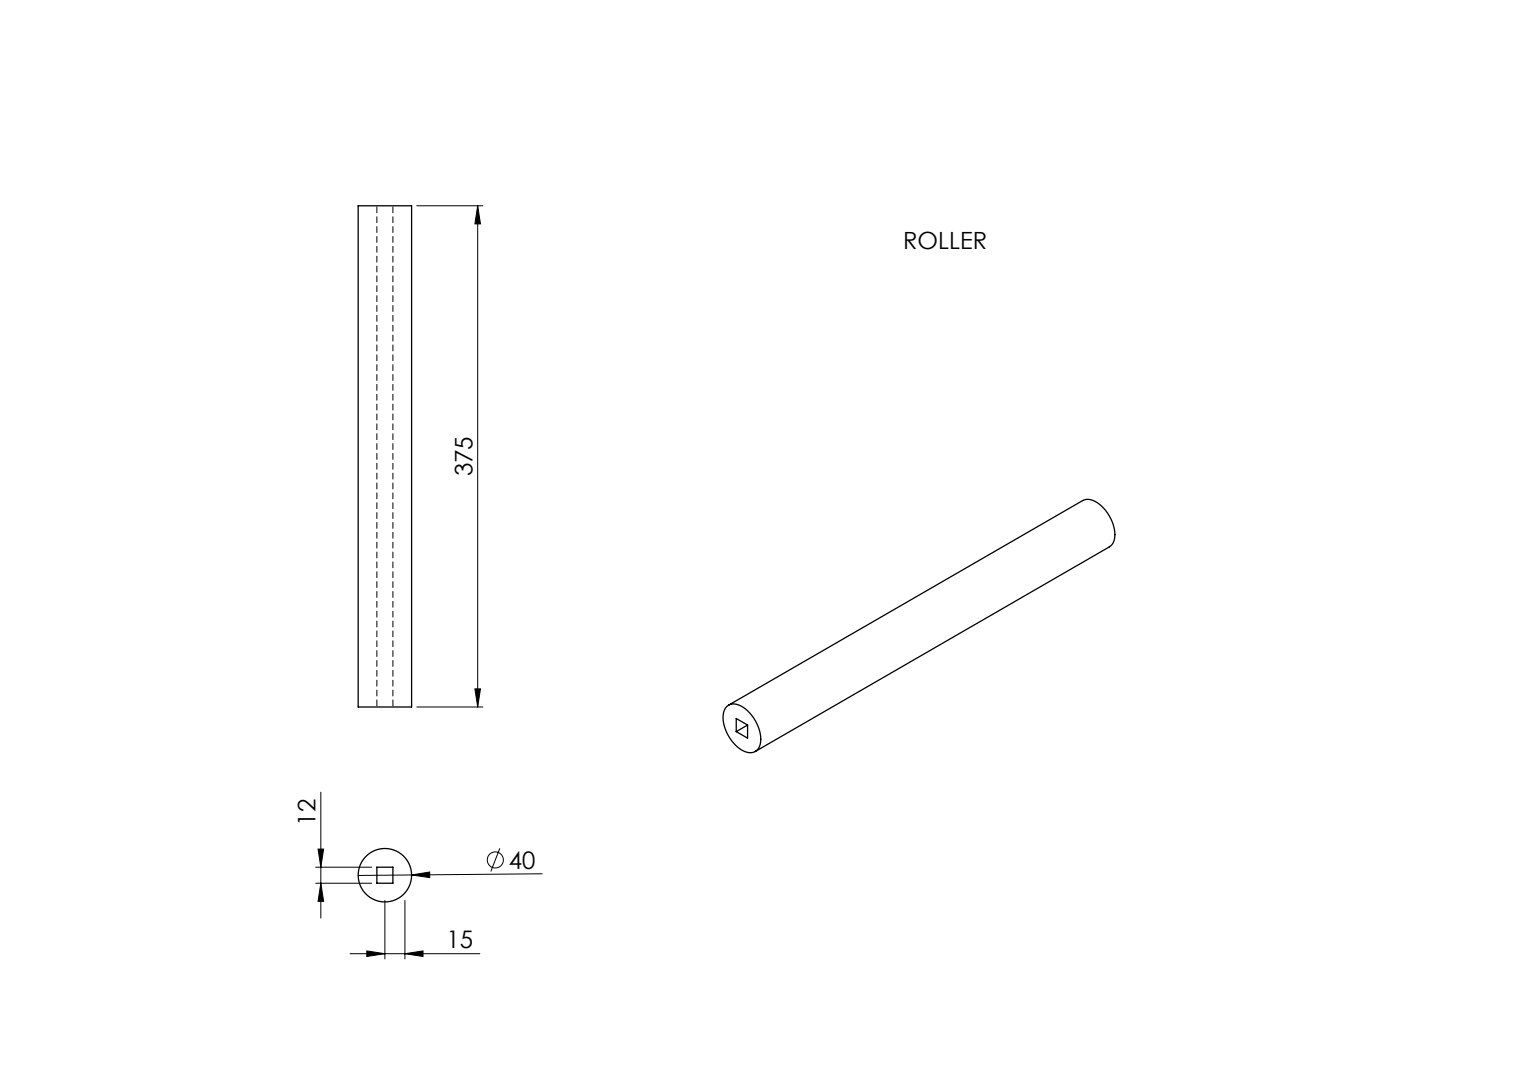
ISO-10303-21;
HEADER;
FILE_DESCRIPTION (('STEP AP214'),
    '1' );
FILE_NAME ('roller.step',
    '2026-10-27T17:01:19',
    ( '' ),
    ( '' ),
    'SwSTEP 2.0',
    'SolidWorks 2026',
    '' );
FILE_SCHEMA (( 'AUTOMOTIVE_DESIGN' ));
ENDSEC;

DATA;
#127=UNCERTAINTY_MEASURE_WITH_UNIT (LENGTH_MEASURE( 1.000000000000000082E-05 ), #3308, 'distance_accuracy_value', 'NONE');
#224=ORIENTED_EDGE ( 'NONE', *, *, #3254, .F. ) ;
#239=LINE ( 'NONE', #9271, #6395 ) ;
#289=LINE ( 'NONE', #6055, #6795 ) ;
#485=COLOUR_RGB ( '',0.8941176470588234615, 0.8941176470588234615, 0.8941176470588234615 ) ;
#555=( LENGTH_UNIT ( ) NAMED_UNIT ( * ) SI_UNIT ( .MILLI., .METRE. ) );
#581=FACE_OUTER_BOUND ( 'NONE', #7020, .T. ) ;
#652=VECTOR ( 'NONE', #13320, 1000.000000000000000 ) ;
#738=CARTESIAN_POINT ( 'NONE',  ( 629.0000000000000000, 166.0000000000000284, -187.5000000000000000 ) ) ;
#787=ADVANCED_FACE ( 'NONE', ( #1021 ), #12234, .F. ) ;
#802=ORIENTED_EDGE ( 'NONE', *, *, #4595, .T. ) ;
#910=DIRECTION ( 'NONE',  ( 1.000000000000000000, 0.000000000000000000, -0.000000000000000000 ) ) ;
#952=FACE_OUTER_BOUND ( 'NONE', #13047, .T. ) ;
#1005=VERTEX_POINT ( 'NONE', #7868 ) ;
#1021=FACE_OUTER_BOUND ( 'NONE', #9658, .T. ) ;
#1036=EDGE_CURVE ( 'NONE', #5493, #9344, #11865, .T. ) ;
#1074=EDGE_CURVE ( 'NONE', #10137, #7536, #3365, .T. ) ;
#1095=EDGE_LOOP ( 'NONE', ( #8108, #3138 ) ) ;
#1160=MECHANICAL_DESIGN_GEOMETRIC_PRESENTATION_REPRESENTATION('',(#3274),#2339);
#1340=EDGE_CURVE ( 'NONE', #10717, #8233, #11743, .T. ) ;
#1404=EDGE_CURVE ( 'NONE', #5419, #13232, #3263, .T. ) ;
#1435=DIRECTION ( 'NONE',  ( 0.000000000000000000, 0.000000000000000000, 1.000000000000000000 ) ) ;
#1567=CARTESIAN_POINT ( 'NONE',  ( 629.0000000000000000, 166.0000000000000284, -187.5000000000000000 ) ) ;
#1672=( NAMED_UNIT ( * ) PLANE_ANGLE_UNIT ( ) SI_UNIT ( $, .RADIAN. ) );
#1675=STYLED_ITEM ( 'NONE', ( #7137 ), #11811 ) ;
#1762=ADVANCED_FACE ( 'NONE', ( #581 ), #13002, .F. ) ;
#1918=AXIS2_PLACEMENT_3D ( 'NONE', #7664, #12083, #13271 ) ;
#2081=VECTOR ( 'NONE', #9838, 1000.000000000000000 ) ;
#2106=CIRCLE ( 'NONE', #7547, 20.00000000000001776 ) ;
#2141=CARTESIAN_POINT ( 'NONE',  ( 629.0000000000000000, 154.0000000000000284, -187.5000000000000000 ) ) ;
#2192=ORIENTED_EDGE ( 'NONE', *, *, #7150, .F. ) ;
#2193=LINE ( 'NONE', #8778, #9880 ) ;
#2339=( GEOMETRIC_REPRESENTATION_CONTEXT ( 3 ) GLOBAL_UNCERTAINTY_ASSIGNED_CONTEXT ( ( #127 ) ) GLOBAL_UNIT_ASSIGNED_CONTEXT ( ( #3308, #11048, #11129 ) ) REPRESENTATION_CONTEXT ( 'NONE', 'WORKASPACE' ) );
#2640=SURFACE_SIDE_STYLE ('',( #6100 ) ) ;
#2690=PLANE ( 'NONE',  #9377 ) ;
#2691=EDGE_LOOP ( 'NONE', ( #13364, #12574, #13404, #8767 ) ) ;
#2702=FACE_OUTER_BOUND ( 'NONE', #2691, .T. ) ;
#2740=CARTESIAN_POINT ( 'NONE',  ( 641.0000000000000000, 154.0000000000000568, -187.5000000000000000 ) ) ;
#2802=CARTESIAN_POINT ( 'NONE',  ( 655.0000000000000000, 160.0000000000000284, 187.5000000000000000 ) ) ;
#2807=UNCERTAINTY_MEASURE_WITH_UNIT (LENGTH_MEASURE( 1.000000000000000082E-05 ), #555, 'distance_accuracy_value', 'NONE');
#2861=ADVANCED_FACE ( 'NONE', ( #9810 ), #14526, .T. ) ;
#2905=PRODUCT ( 'roller', 'roller', '', ( #8858 ) ) ;
#3031=AXIS2_PLACEMENT_3D ( 'NONE', #3787, #3708, #7309 ) ;
#3105=DIRECTION ( 'NONE',  ( -0.000000000000000000, -0.000000000000000000, 1.000000000000000000 ) ) ;
#3138=ORIENTED_EDGE ( 'NONE', *, *, #13421, .F. ) ;
#3242=CARTESIAN_POINT ( 'NONE',  ( 641.0000000000000000, 154.0000000000000568, -187.5000000000000000 ) ) ;
#3254=EDGE_CURVE ( 'NONE', #7536, #5493, #9993, .T. ) ;
#3263=LINE ( 'NONE', #8654, #8679 ) ;
#3274=STYLED_ITEM('',(#14667),#7155);
#3308=( LENGTH_UNIT ( ) NAMED_UNIT ( * ) SI_UNIT ( .MILLI., .METRE. ) );
#3318=VECTOR ( 'NONE', #5866, 1000.000000000000000 ) ;
#3365=LINE ( 'NONE', #14442, #652 ) ;
#3459=DIRECTION ( 'NONE',  ( 1.000000000000000000, -0.000000000000000000, 0.000000000000000000 ) ) ;
#3514=ADVANCED_FACE ( 'NONE', ( #5114, #12110 ), #14049, .F. ) ;
#3594=CARTESIAN_POINT ( 'NONE',  ( 635.0000000000000000, 160.0000000000000284, 187.5000000000000000 ) ) ;
#3683=EDGE_CURVE ( 'NONE', #8233, #5419, #9901, .T. ) ;
#3708=DIRECTION ( 'NONE',  ( -0.000000000000000000, 1.000000000000000000, 0.000000000000000000 ) ) ;
#3731=CARTESIAN_POINT ( 'NONE',  ( 615.0000000000000000, 160.0000000000000284, 187.5000000000000000 ) ) ;
#3765=AXIS2_PLACEMENT_3D ( 'NONE', #7403, #6282, #5184 ) ;
#3782=VECTOR ( 'NONE', #11666, 1000.000000000000000 ) ;
#3787=CARTESIAN_POINT ( 'NONE',  ( 629.0000000000000000, 166.0000000000000284, -187.5000000000000000 ) ) ;
#3906=CARTESIAN_POINT ( 'NONE',  ( 615.0000000000000000, 160.0000000000000284, -187.5000000000000000 ) ) ;
#3983=AXIS2_PLACEMENT_3D ( 'NONE', #13343, #4416, #13417 ) ;
#4086=ORIENTED_EDGE ( 'NONE', *, *, #1036, .F. ) ;
#4092=AXIS2_PLACEMENT_3D ( 'NONE', #9935, #7491, #910 ) ;
#4219=ORIENTED_EDGE ( 'NONE', *, *, #6873, .F. ) ;
#4347=CARTESIAN_POINT ( 'NONE',  ( 0.000000000000000000, 0.000000000000000000, 0.000000000000000000 ) ) ;
#4416=DIRECTION ( 'NONE',  ( -0.000000000000000000, -0.000000000000000000, -1.000000000000000000 ) ) ;
#4431=DIRECTION ( 'NONE',  ( 1.000000000000000000, 0.000000000000000000, 0.000000000000000000 ) ) ;
#4595=EDGE_CURVE ( 'NONE', #10717, #7536, #9195, .T. ) ;
#4719=CIRCLE ( 'NONE', #11998, 20.00000000000001776 ) ;
#4791=FILL_AREA_STYLE_COLOUR ( '', #485 ) ;
#4995=ORIENTED_EDGE ( 'NONE', *, *, #8442, .T. ) ;
#5040=PRODUCT_DEFINITION_CONTEXT ( 'detailed design', #10844, 'design' ) ;
#5092=VERTEX_POINT ( 'NONE', #2802 ) ;
#5114=FACE_BOUND ( 'NONE', #13576, .T. ) ;
#5150=CARTESIAN_POINT ( 'NONE',  ( 629.0000000000000000, 154.0000000000000284, -187.5000000000000000 ) ) ;
#5184=DIRECTION ( 'NONE',  ( 1.000000000000000000, 0.000000000000000000, -0.000000000000000000 ) ) ;
#5192=ORIENTED_EDGE ( 'NONE', *, *, #12792, .F. ) ;
#5376=ORIENTED_EDGE ( 'NONE', *, *, #1074, .T. ) ;
#5419=VERTEX_POINT ( 'NONE', #5150 ) ;
#5433=PLANE ( 'NONE',  #4092 ) ;
#5450=( GEOMETRIC_REPRESENTATION_CONTEXT ( 3 ) GLOBAL_UNCERTAINTY_ASSIGNED_CONTEXT ( ( #2807 ) ) GLOBAL_UNIT_ASSIGNED_CONTEXT ( ( #555, #1672, #6246 ) ) REPRESENTATION_CONTEXT ( 'NONE', 'WORKASPACE' ) );
#5487=VERTEX_POINT ( 'NONE', #3906 ) ;
#5493=VERTEX_POINT ( 'NONE', #8388 ) ;
#5706=EDGE_LOOP ( 'NONE', ( #2192, #8047, #9060, #11679 ) ) ;
#5866=DIRECTION ( 'NONE',  ( -0.000000000000000000, -0.000000000000000000, 1.000000000000000000 ) ) ;
#5911=AXIS2_PLACEMENT_3D ( 'NONE', #6575, #14539, #4431 ) ;
#5926=CARTESIAN_POINT ( 'NONE',  ( 641.0000000000000000, 154.0000000000000568, -187.5000000000000000 ) ) ;
#5945=ORIENTED_EDGE ( 'NONE', *, *, #9374, .T. ) ;
#6055=CARTESIAN_POINT ( 'NONE',  ( 615.0000000000000000, 160.0000000000000284, 187.5000000000000000 ) ) ;
#6077=DIRECTION ( 'NONE',  ( -1.000000000000000000, -0.000000000000000000, -0.000000000000000000 ) ) ;
#6100=SURFACE_STYLE_FILL_AREA ( #12660 ) ;
#6246=( NAMED_UNIT ( * ) SI_UNIT ( $, .STERADIAN. ) SOLID_ANGLE_UNIT ( ) );
#6282=DIRECTION ( 'NONE',  ( 0.000000000000000000, 0.000000000000000000, 1.000000000000000000 ) ) ;
#6328=VECTOR ( 'NONE', #12276, 1000.000000000000000 ) ;
#6331=CARTESIAN_POINT ( 'NONE',  ( 635.0000000000000000, 160.0000000000000284, -187.5000000000000000 ) ) ;
#6395=VECTOR ( 'NONE', #8973, 1000.000000000000000 ) ;
#6417=DIRECTION ( 'NONE',  ( 1.000000000000000000, 0.000000000000000000, 0.000000000000000000 ) ) ;
#6575=CARTESIAN_POINT ( 'NONE',  ( 635.0000000000000000, 160.0000000000000284, -187.5000000000000000 ) ) ;
#6609=FACE_BOUND ( 'NONE', #12156, .T. ) ;
#6643=AXIS2_PLACEMENT_3D ( 'NONE', #13841, #9501, #11690 ) ;
#6660=DIRECTION ( 'NONE',  ( -0.000000000000000000, -1.000000000000000000, -0.000000000000000000 ) ) ;
#6664=ADVANCED_FACE ( 'NONE', ( #13829 ), #2690, .F. ) ;
#6693=ORIENTED_EDGE ( 'NONE', *, *, #9359, .F. ) ;
#6718=CYLINDRICAL_SURFACE ( 'NONE', #13445, 20.00000000000001776 ) ;
#6786=VECTOR ( 'NONE', #6077, 1000.000000000000000 ) ;
#6795=VECTOR ( 'NONE', #13814, 1000.000000000000000 ) ;
#6821=ORIENTED_EDGE ( 'NONE', *, *, #1404, .T. ) ;
#6849=CIRCLE ( 'NONE', #5911, 20.00000000000001776 ) ;
#6853=( GEOMETRIC_REPRESENTATION_CONTEXT ( 3 ) GLOBAL_UNCERTAINTY_ASSIGNED_CONTEXT ( ( #10337 ) ) GLOBAL_UNIT_ASSIGNED_CONTEXT ( ( #8018, #12963, #7206 ) ) REPRESENTATION_CONTEXT ( 'NONE', 'WORKASPACE' ) );
#6873=EDGE_CURVE ( 'NONE', #9344, #10137, #7555, .T. ) ;
#6959=SHAPE_REPRESENTATION ( 'roller', ( #9440 ), #6853 ) ;
#7020=EDGE_LOOP ( 'NONE', ( #13518, #10734, #802, #11658 ) ) ;
#7137=PRESENTATION_STYLE_ASSIGNMENT (( #10679 ) ) ;
#7147=CLOSED_SHELL ( 'NONE', ( #2861, #8345, #12139, #3514, #787, #10970, #6664, #1762 ) ) ;
#7150=EDGE_CURVE ( 'NONE', #5419, #9344, #2193, .T. ) ;
#7155=MANIFOLD_SOLID_BREP ( 'Cut-Extrude1', #7147 ) ;
#7177=LINE ( 'NONE', #5926, #3782 ) ;
#7187=CARTESIAN_POINT ( 'NONE',  ( 629.0000000000000000, 154.0000000000000284, -187.5000000000000000 ) ) ;
#7206=( NAMED_UNIT ( * ) SI_UNIT ( $, .STERADIAN. ) SOLID_ANGLE_UNIT ( ) );
#7309=DIRECTION ( 'NONE',  ( 0.000000000000000000, -0.000000000000000000, 1.000000000000000000 ) ) ;
#7403=CARTESIAN_POINT ( 'NONE',  ( 635.0000000000000000, 160.0000000000000284, -187.5000000000000000 ) ) ;
#7472=EDGE_CURVE ( 'NONE', #5092, #7639, #2106, .T. ) ;
#7491=DIRECTION ( 'NONE',  ( 0.000000000000000000, 0.000000000000000000, 1.000000000000000000 ) ) ;
#7495=CARTESIAN_POINT ( 'NONE',  ( 641.0000000000000000, 154.0000000000000568, -187.5000000000000000 ) ) ;
#7511=ORIENTED_EDGE ( 'NONE', *, *, #12792, .T. ) ;
#7536=VERTEX_POINT ( 'NONE', #12583 ) ;
#7547=AXIS2_PLACEMENT_3D ( 'NONE', #3594, #7795, #13546 ) ;
#7555=LINE ( 'NONE', #13160, #2081 ) ;
#7570=VECTOR ( 'NONE', #3105, 1000.000000000000000 ) ;
#7591=DIRECTION ( 'NONE',  ( 1.000000000000000000, 0.000000000000000000, 0.000000000000000000 ) ) ;
#7608=PRODUCT_DEFINITION_SHAPE ( 'NONE', 'NONE',  #8184 ) ;
#7639=VERTEX_POINT ( 'NONE', #3731 ) ;
#7664=CARTESIAN_POINT ( 'NONE',  ( 635.0000000000000000, 160.0000000000000284, 187.5000000000000000 ) ) ;
#7696=DIRECTION ( 'NONE',  ( 1.000000000000000000, 2.312964634635740689E-15, 0.000000000000000000 ) ) ;
#7708=ORIENTED_EDGE ( 'NONE', *, *, #3683, .T. ) ;
#7729=DIRECTION ( 'NONE',  ( 0.000000000000000000, 0.000000000000000000, 1.000000000000000000 ) ) ;
#7756=DIRECTION ( 'NONE',  ( -0.000000000000000000, -0.000000000000000000, -1.000000000000000000 ) ) ;
#7795=DIRECTION ( 'NONE',  ( 0.000000000000000000, 0.000000000000000000, 1.000000000000000000 ) ) ;
#7824=LINE ( 'NONE', #9815, #7570 ) ;
#7864=EDGE_LOOP ( 'NONE', ( #10203, #14277 ) ) ;
#7868=CARTESIAN_POINT ( 'NONE',  ( 655.0000000000000000, 160.0000000000000284, -187.5000000000000000 ) ) ;
#7896=DIRECTION ( 'NONE',  ( 0.000000000000000000, 0.000000000000000000, -1.000000000000000000 ) ) ;
#7937=CARTESIAN_POINT ( 'NONE',  ( 641.0000000000000000, 166.0000000000000284, -187.5000000000000000 ) ) ;
#8018=( LENGTH_UNIT ( ) NAMED_UNIT ( * ) SI_UNIT ( .MILLI., .METRE. ) );
#8047=ORIENTED_EDGE ( 'NONE', *, *, #3683, .F. ) ;
#8108=ORIENTED_EDGE ( 'NONE', *, *, #8442, .F. ) ;
#8137=DIRECTION ( 'NONE',  ( -1.000000000000000000, 0.000000000000000000, 0.000000000000000000 ) ) ;
#8184=PRODUCT_DEFINITION ( 'UNKNOWN', '', #10199, #5040 ) ;
#8214=VECTOR ( 'NONE', #11388, 1000.000000000000000 ) ;
#8233=VERTEX_POINT ( 'NONE', #738 ) ;
#8345=ADVANCED_FACE ( 'NONE', ( #952 ), #6718, .T. ) ;
#8388=CARTESIAN_POINT ( 'NONE',  ( 629.0000000000000000, 166.0000000000000284, 187.5000000000000000 ) ) ;
#8416=ORIENTED_EDGE ( 'NONE', *, *, #7472, .F. ) ;
#8442=EDGE_CURVE ( 'NONE', #5487, #1005, #6849, .T. ) ;
#8620=ORIENTED_EDGE ( 'NONE', *, *, #8848, .T. ) ;
#8654=CARTESIAN_POINT ( 'NONE',  ( 629.0000000000000000, 154.0000000000000284, -187.5000000000000000 ) ) ;
#8679=VECTOR ( 'NONE', #7696, 1000.000000000000000 ) ;
#8694=DIRECTION ( 'NONE',  ( -0.000000000000000000, -0.000000000000000000, 1.000000000000000000 ) ) ;
#8767=ORIENTED_EDGE ( 'NONE', *, *, #6873, .T. ) ;
#8778=CARTESIAN_POINT ( 'NONE',  ( 629.0000000000000000, 154.0000000000000284, -187.5000000000000000 ) ) ;
#8848=EDGE_CURVE ( 'NONE', #5092, #1005, #239, .T. ) ;
#8858=PRODUCT_CONTEXT ( 'NONE', #12344, 'mechanical' ) ;
#8973=DIRECTION ( 'NONE',  ( -0.000000000000000000, -0.000000000000000000, -1.000000000000000000 ) ) ;
#9060=ORIENTED_EDGE ( 'NONE', *, *, #10355, .T. ) ;
#9146=DIRECTION ( 'NONE',  ( -1.000000000000000000, 0.000000000000000000, 0.000000000000000000 ) ) ;
#9195=LINE ( 'NONE', #7937, #3318 ) ;
#9271=CARTESIAN_POINT ( 'NONE',  ( 655.0000000000000000, 160.0000000000000284, 187.5000000000000000 ) ) ;
#9323=CARTESIAN_POINT ( 'NONE',  ( 629.0000000000000000, 154.0000000000000284, 187.5000000000000000 ) ) ;
#9344=VERTEX_POINT ( 'NONE', #9323 ) ;
#9359=EDGE_CURVE ( 'NONE', #13232, #10717, #7177, .T. ) ;
#9374=EDGE_CURVE ( 'NONE', #13232, #10137, #12710, .T. ) ;
#9377=AXIS2_PLACEMENT_3D ( 'NONE', #7187, #8137, #1435 ) ;
#9440=AXIS2_PLACEMENT_3D ( 'NONE', #4347, #14302, #6417 ) ;
#9501=DIRECTION ( 'NONE',  ( 2.312964634635740689E-15, -1.000000000000000000, 0.000000000000000000 ) ) ;
#9658=EDGE_LOOP ( 'NONE', ( #9716, #6693, #5945, #5376 ) ) ;
#9716=ORIENTED_EDGE ( 'NONE', *, *, #4595, .F. ) ;
#9810=FACE_OUTER_BOUND ( 'NONE', #14045, .T. ) ;
#9815=CARTESIAN_POINT ( 'NONE',  ( 629.0000000000000000, 166.0000000000000284, -187.5000000000000000 ) ) ;
#9838=DIRECTION ( 'NONE',  ( 1.000000000000000000, 2.312964634635740689E-15, 0.000000000000000000 ) ) ;
#9868=CARTESIAN_POINT ( 'NONE',  ( 641.0000000000000000, 166.0000000000000284, -187.5000000000000000 ) ) ;
#9880=VECTOR ( 'NONE', #8694, 1000.000000000000000 ) ;
#9901=LINE ( 'NONE', #2141, #13897 ) ;
#9935=CARTESIAN_POINT ( 'NONE',  ( 635.0000000000000000, 160.0000000000000284, 187.5000000000000000 ) ) ;
#9993=LINE ( 'NONE', #10212, #8214 ) ;
#10137=VERTEX_POINT ( 'NONE', #14033 ) ;
#10154=MECHANICAL_DESIGN_GEOMETRIC_PRESENTATION_REPRESENTATION('',(#1675),#5450);
#10170=ORIENTED_EDGE ( 'NONE', *, *, #9359, .T. ) ;
#10199=PRODUCT_DEFINITION_FORMATION_WITH_SPECIFIED_SOURCE ( 'ANY', '', #2905, .NOT_KNOWN. ) ;
#10203=ORIENTED_EDGE ( 'NONE', *, *, #10687, .T. ) ;
#10212=CARTESIAN_POINT ( 'NONE',  ( 629.0000000000000000, 166.0000000000000284, 187.5000000000000000 ) ) ;
#10245=AXIS2_PLACEMENT_3D ( 'NONE', #3242, #3459, #7896 ) ;
#10337=UNCERTAINTY_MEASURE_WITH_UNIT (LENGTH_MEASURE( 1.000000000000000082E-05 ), #8018, 'distance_accuracy_value', 'NONE');
#10355=EDGE_CURVE ( 'NONE', #8233, #5493, #7824, .T. ) ;
#10679=SURFACE_STYLE_USAGE ( .BOTH. , #2640 ) ;
#10687=EDGE_CURVE ( 'NONE', #7639, #5092, #11348, .T. ) ;
#10690=ORIENTED_EDGE ( 'NONE', *, *, #1074, .F. ) ;
#10717=VERTEX_POINT ( 'NONE', #9868 ) ;
#10734=ORIENTED_EDGE ( 'NONE', *, *, #1340, .F. ) ;
#10745=ORIENTED_EDGE ( 'NONE', *, *, #13421, .T. ) ;
#10844=APPLICATION_CONTEXT ( 'automotive_design' ) ;
#10970=ADVANCED_FACE ( 'NONE', ( #2702 ), #12959, .F. ) ;
#11048=( NAMED_UNIT ( * ) PLANE_ANGLE_UNIT ( ) SI_UNIT ( $, .RADIAN. ) );
#11129=( NAMED_UNIT ( * ) SI_UNIT ( $, .STERADIAN. ) SOLID_ANGLE_UNIT ( ) );
#11291=ORIENTED_EDGE ( 'NONE', *, *, #1340, .T. ) ;
#11348=CIRCLE ( 'NONE', #1918, 20.00000000000001776 ) ;
#11388=DIRECTION ( 'NONE',  ( -1.000000000000000000, -0.000000000000000000, -0.000000000000000000 ) ) ;
#11658=ORIENTED_EDGE ( 'NONE', *, *, #3254, .T. ) ;
#11666=DIRECTION ( 'NONE',  ( 0.000000000000000000, 1.000000000000000000, 0.000000000000000000 ) ) ;
#11679=ORIENTED_EDGE ( 'NONE', *, *, #1036, .T. ) ;
#11690=DIRECTION ( 'NONE',  ( 1.000000000000000000, 2.312964634635740689E-15, 0.000000000000000000 ) ) ;
#11694=SHAPE_REPRESENTATION_RELATIONSHIP ( 'NONE' , 'NONE' ,  #6959, #11811 ) ;
#11743=LINE ( 'NONE', #1567, #6786 ) ;
#11811=ADVANCED_BREP_SHAPE_REPRESENTATION ( '', ( #7155, #9440 ), #6853 ) ;
#11865=LINE ( 'NONE', #12351, #6328 ) ;
#11998=AXIS2_PLACEMENT_3D ( 'NONE', #6331, #7729, #7591 ) ;
#12013=VECTOR ( 'NONE', #12636, 1000.000000000000000 ) ;
#12083=DIRECTION ( 'NONE',  ( 0.000000000000000000, 0.000000000000000000, 1.000000000000000000 ) ) ;
#12110=FACE_OUTER_BOUND ( 'NONE', #1095, .T. ) ;
#12139=ADVANCED_FACE ( 'NONE', ( #6609, #12198 ), #5433, .T. ) ;
#12156=EDGE_LOOP ( 'NONE', ( #10690, #4219, #4086, #224 ) ) ;
#12198=FACE_OUTER_BOUND ( 'NONE', #7864, .T. ) ;
#12234=PLANE ( 'NONE',  #10245 ) ;
#12276=DIRECTION ( 'NONE',  ( -0.000000000000000000, -1.000000000000000000, -0.000000000000000000 ) ) ;
#12344=APPLICATION_CONTEXT ( 'automotive_design' ) ;
#12351=CARTESIAN_POINT ( 'NONE',  ( 629.0000000000000000, 154.0000000000000284, 187.5000000000000000 ) ) ;
#12574=ORIENTED_EDGE ( 'NONE', *, *, #1404, .F. ) ;
#12583=CARTESIAN_POINT ( 'NONE',  ( 641.0000000000000000, 166.0000000000000284, 187.5000000000000000 ) ) ;
#12615=ORIENTED_EDGE ( 'NONE', *, *, #8848, .F. ) ;
#12636=DIRECTION ( 'NONE',  ( -0.000000000000000000, -0.000000000000000000, 1.000000000000000000 ) ) ;
#12660=FILL_AREA_STYLE ('',( #4791 ) ) ;
#12710=LINE ( 'NONE', #2740, #12013 ) ;
#12792=EDGE_CURVE ( 'NONE', #7639, #5487, #289, .T. ) ;
#12959=PLANE ( 'NONE',  #6643 ) ;
#12963=( NAMED_UNIT ( * ) PLANE_ANGLE_UNIT ( ) SI_UNIT ( $, .RADIAN. ) );
#13002=PLANE ( 'NONE',  #3031 ) ;
#13047=EDGE_LOOP ( 'NONE', ( #12615, #13173, #7511, #4995 ) ) ;
#13160=CARTESIAN_POINT ( 'NONE',  ( 629.0000000000000000, 154.0000000000000284, 187.5000000000000000 ) ) ;
#13173=ORIENTED_EDGE ( 'NONE', *, *, #10687, .F. ) ;
#13232=VERTEX_POINT ( 'NONE', #7495 ) ;
#13271=DIRECTION ( 'NONE',  ( 1.000000000000000000, 0.000000000000000000, 0.000000000000000000 ) ) ;
#13320=DIRECTION ( 'NONE',  ( 0.000000000000000000, 1.000000000000000000, 0.000000000000000000 ) ) ;
#13343=CARTESIAN_POINT ( 'NONE',  ( 635.0000000000000000, 160.0000000000000284, 187.5000000000000000 ) ) ;
#13364=ORIENTED_EDGE ( 'NONE', *, *, #9374, .F. ) ;
#13404=ORIENTED_EDGE ( 'NONE', *, *, #7150, .T. ) ;
#13417=DIRECTION ( 'NONE',  ( -1.000000000000000000, 0.000000000000000000, 0.000000000000000000 ) ) ;
#13421=EDGE_CURVE ( 'NONE', #1005, #5487, #4719, .T. ) ;
#13445=AXIS2_PLACEMENT_3D ( 'NONE', #13515, #7756, #9146 ) ;
#13515=CARTESIAN_POINT ( 'NONE',  ( 635.0000000000000000, 160.0000000000000284, 187.5000000000000000 ) ) ;
#13518=ORIENTED_EDGE ( 'NONE', *, *, #10355, .F. ) ;
#13546=DIRECTION ( 'NONE',  ( 1.000000000000000000, 0.000000000000000000, 0.000000000000000000 ) ) ;
#13576=EDGE_LOOP ( 'NONE', ( #6821, #10170, #11291, #7708 ) ) ;
#13814=DIRECTION ( 'NONE',  ( -0.000000000000000000, -0.000000000000000000, -1.000000000000000000 ) ) ;
#13829=FACE_OUTER_BOUND ( 'NONE', #5706, .T. ) ;
#13841=CARTESIAN_POINT ( 'NONE',  ( 629.0000000000000000, 154.0000000000000284, -187.5000000000000000 ) ) ;
#13897=VECTOR ( 'NONE', #6660, 1000.000000000000000 ) ;
#14033=CARTESIAN_POINT ( 'NONE',  ( 641.0000000000000000, 154.0000000000000568, 187.5000000000000000 ) ) ;
#14045=EDGE_LOOP ( 'NONE', ( #8416, #8620, #10745, #5192 ) ) ;
#14049=PLANE ( 'NONE',  #3765 ) ;
#14277=ORIENTED_EDGE ( 'NONE', *, *, #7472, .T. ) ;
#14302=DIRECTION ( 'NONE',  ( 0.000000000000000000, 0.000000000000000000, 1.000000000000000000 ) ) ;
#14442=CARTESIAN_POINT ( 'NONE',  ( 641.0000000000000000, 154.0000000000000568, 187.5000000000000000 ) ) ;
#14526=CYLINDRICAL_SURFACE ( 'NONE', #3983, 20.00000000000001776 ) ;
#14538=SHAPE_DEFINITION_REPRESENTATION ( #7608, #6959 ) ;
#14539=DIRECTION ( 'NONE',  ( 0.000000000000000000, 0.000000000000000000, 1.000000000000000000 ) ) ;
#14661=COLOUR_RGB('Sky Blue',0.24,0.69,0.87);
#14662=FILL_AREA_STYLE_COLOUR('',#14661);
#14663=FILL_AREA_STYLE('',(#14662));
#14664=SURFACE_STYLE_FILL_AREA(#14663);
#14665=SURFACE_SIDE_STYLE('',(#14664));
#14666=SURFACE_STYLE_USAGE(.BOTH.,#14665);
#14667=PRESENTATION_STYLE_ASSIGNMENT((#14666));
ENDSEC;
END-ISO-10303-21;
